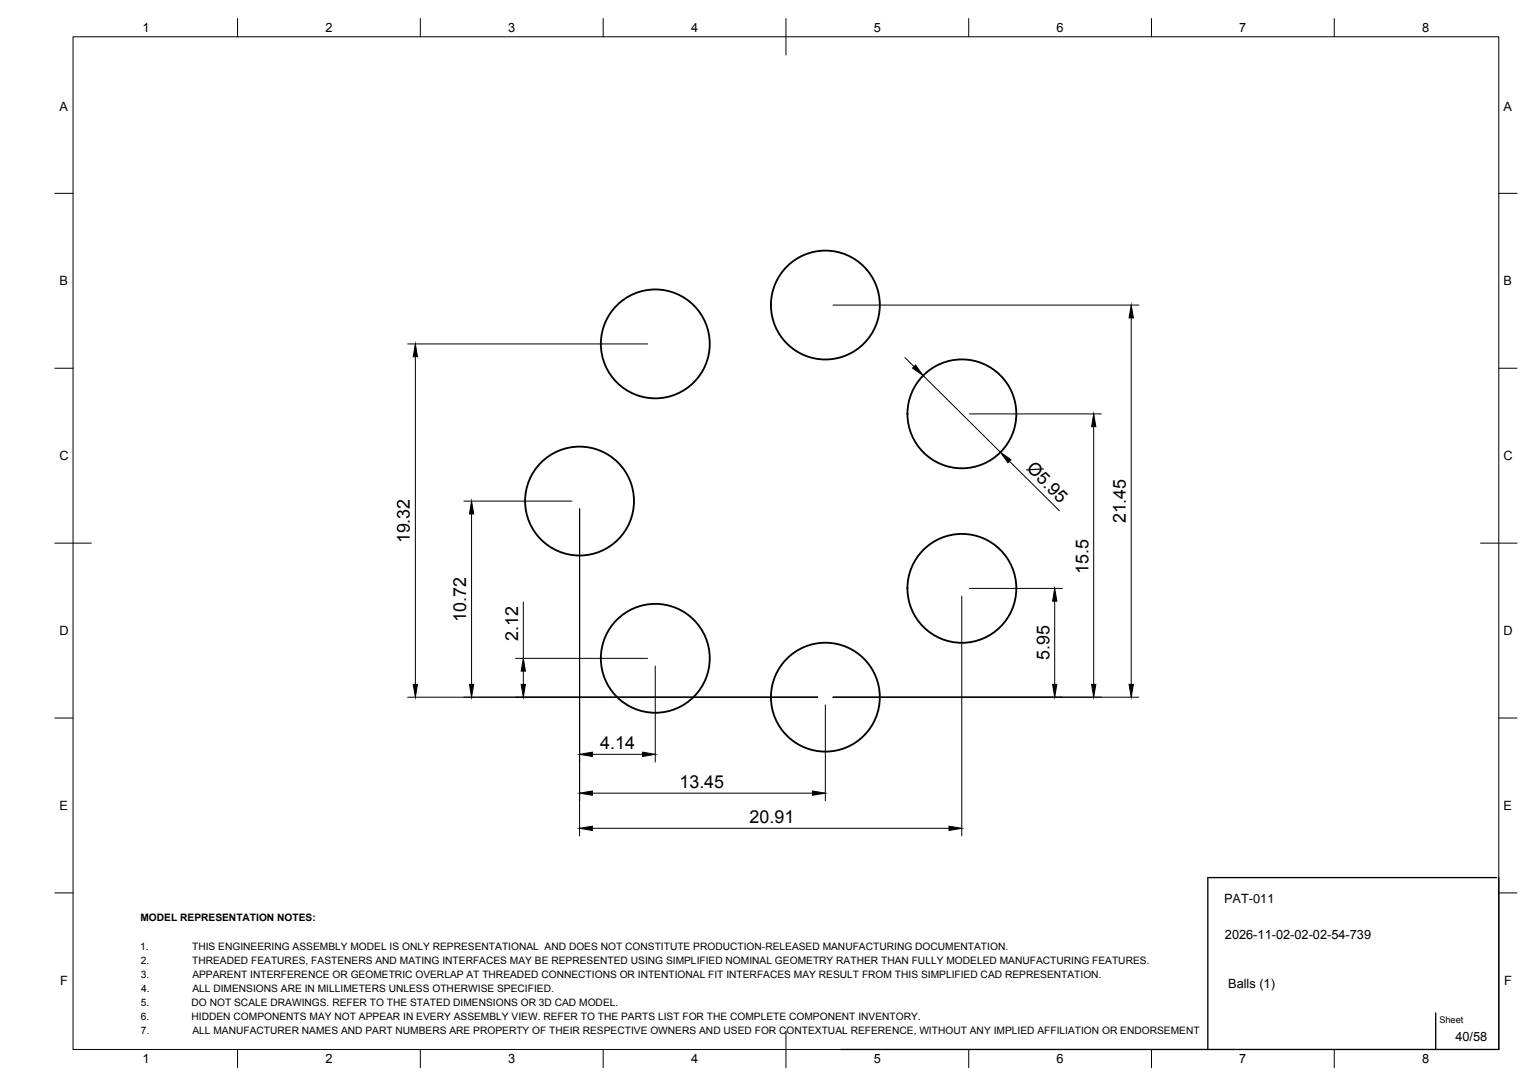
ISO-10303-21;
HEADER;
/* Generated by software containing ST-Developer
 * from STEP Tools, Inc. (www.steptools.com) 
 */

FILE_DESCRIPTION(
/* description */ ('Belt tension measurement rig'),
/* implementation_level */ '2;1');

FILE_NAME(
/* name */ 'Balls (1).step',
/* time_stamp */ '2026-10-28T03:24:44-07:00',
/* author */ (''),
/* organization */ (''),
/* preprocessor_version */ 'ST-DEVELOPER v20.2',
/* originating_system */ 'Autodesk Translation Framework v15.17.0.0',
/* authorisation */ '');

FILE_SCHEMA (('AUTOMOTIVE_DESIGN { 1 0 10303 214 3 1 1 }'));
ENDSEC;

DATA;
#10=MECHANICAL_DESIGN_GEOMETRIC_PRESENTATION_REPRESENTATION('',(#733,#734,#735,#736,#737,#738,#739),#23587);
#453=SPHERICAL_SURFACE('',#13695,0.29765);
#454=SPHERICAL_SURFACE('',#13697,0.29765);
#455=SPHERICAL_SURFACE('',#13699,0.29765);
#456=SPHERICAL_SURFACE('',#13701,0.29765);
#457=SPHERICAL_SURFACE('',#13703,0.29765);
#458=SPHERICAL_SURFACE('',#13705,0.29765);
#459=SPHERICAL_SURFACE('',#13707,0.29765);
#615=SHAPE_REPRESENTATION_RELATIONSHIP('SRR','None',#23864,#670);
#670=ADVANCED_BREP_SHAPE_REPRESENTATION('',(#802,#803,#804,#805,#806,#807,
#808),#23562);
#733=STYLED_ITEM('',(#24211),#802);
#734=STYLED_ITEM('',(#24211),#803);
#735=STYLED_ITEM('',(#24211),#804);
#736=STYLED_ITEM('',(#24211),#805);
#737=STYLED_ITEM('',(#24211),#806);
#738=STYLED_ITEM('',(#24211),#807);
#739=STYLED_ITEM('',(#24211),#808);
#802=MANIFOLD_SOLID_BREP('Body1',#12239);
#803=MANIFOLD_SOLID_BREP('Body2',#12240);
#804=MANIFOLD_SOLID_BREP('Body3',#12241);
#805=MANIFOLD_SOLID_BREP('Body4',#12242);
#806=MANIFOLD_SOLID_BREP('Body5',#12243);
#807=MANIFOLD_SOLID_BREP('Body6',#12244);
#808=MANIFOLD_SOLID_BREP('Body7',#12245);
#1751=FACE_OUTER_BOUND('',#2604,.T.);
#1752=FACE_OUTER_BOUND('',#2605,.T.);
#1753=FACE_OUTER_BOUND('',#2606,.T.);
#1754=FACE_OUTER_BOUND('',#2607,.T.);
#1755=FACE_OUTER_BOUND('',#2608,.T.);
#1756=FACE_OUTER_BOUND('',#2609,.T.);
#1757=FACE_OUTER_BOUND('',#2610,.T.);
#2604=EDGE_LOOP('',(#9726,#9727));
#2605=EDGE_LOOP('',(#9728,#9729));
#2606=EDGE_LOOP('',(#9730,#9731));
#2607=EDGE_LOOP('',(#9732,#9733));
#2608=EDGE_LOOP('',(#9734,#9735));
#2609=EDGE_LOOP('',(#9736,#9737));
#2610=EDGE_LOOP('',(#9738,#9739));
#4842=CIRCLE('',#13696,0.29765);
#4843=CIRCLE('',#13698,0.29765);
#4844=CIRCLE('',#13700,0.29765);
#4845=CIRCLE('',#13702,0.29765);
#4846=CIRCLE('',#13704,0.29765);
#4847=CIRCLE('',#13706,0.29765);
#4848=CIRCLE('',#13708,0.29765);
#5838=VERTEX_POINT('',#20922);
#5839=VERTEX_POINT('',#20923);
#5840=VERTEX_POINT('',#20926);
#5841=VERTEX_POINT('',#20927);
#5842=VERTEX_POINT('',#20930);
#5843=VERTEX_POINT('',#20931);
#5844=VERTEX_POINT('',#20934);
#5845=VERTEX_POINT('',#20935);
#5846=VERTEX_POINT('',#20938);
#5847=VERTEX_POINT('',#20939);
#5848=VERTEX_POINT('',#20942);
#5849=VERTEX_POINT('',#20943);
#5850=VERTEX_POINT('',#20946);
#5851=VERTEX_POINT('',#20947);
#7222=EDGE_CURVE('',#5838,#5839,#4842,.T.);
#7223=EDGE_CURVE('',#5840,#5841,#4843,.T.);
#7224=EDGE_CURVE('',#5842,#5843,#4844,.T.);
#7225=EDGE_CURVE('',#5844,#5845,#4845,.T.);
#7226=EDGE_CURVE('',#5846,#5847,#4846,.T.);
#7227=EDGE_CURVE('',#5848,#5849,#4847,.T.);
#7228=EDGE_CURVE('',#5850,#5851,#4848,.T.);
#9726=ORIENTED_EDGE('',*,*,#7222,.T.);
#9727=ORIENTED_EDGE('',*,*,#7222,.F.);
#9728=ORIENTED_EDGE('',*,*,#7223,.T.);
#9729=ORIENTED_EDGE('',*,*,#7223,.F.);
#9730=ORIENTED_EDGE('',*,*,#7224,.T.);
#9731=ORIENTED_EDGE('',*,*,#7224,.F.);
#9732=ORIENTED_EDGE('',*,*,#7225,.T.);
#9733=ORIENTED_EDGE('',*,*,#7225,.F.);
#9734=ORIENTED_EDGE('',*,*,#7226,.T.);
#9735=ORIENTED_EDGE('',*,*,#7226,.F.);
#9736=ORIENTED_EDGE('',*,*,#7227,.T.);
#9737=ORIENTED_EDGE('',*,*,#7227,.F.);
#9738=ORIENTED_EDGE('',*,*,#7228,.T.);
#9739=ORIENTED_EDGE('',*,*,#7228,.F.);
#11892=ADVANCED_FACE('',(#1751),#453,.T.);
#11893=ADVANCED_FACE('',(#1752),#454,.T.);
#11894=ADVANCED_FACE('',(#1753),#455,.T.);
#11895=ADVANCED_FACE('',(#1754),#456,.T.);
#11896=ADVANCED_FACE('',(#1755),#457,.T.);
#11897=ADVANCED_FACE('',(#1756),#458,.T.);
#11898=ADVANCED_FACE('',(#1757),#459,.T.);
#12239=CLOSED_SHELL('',(#11892));
#12240=CLOSED_SHELL('',(#11893));
#12241=CLOSED_SHELL('',(#11894));
#12242=CLOSED_SHELL('',(#11895));
#12243=CLOSED_SHELL('',(#11896));
#12244=CLOSED_SHELL('',(#11897));
#12245=CLOSED_SHELL('',(#11898));
#13694=AXIS2_PLACEMENT_3D('',#20920,#16649,#16650);
#13695=AXIS2_PLACEMENT_3D('',#20921,#16651,#16652);
#13696=AXIS2_PLACEMENT_3D('',#20924,#16653,#16654);
#13697=AXIS2_PLACEMENT_3D('',#20925,#16655,#16656);
#13698=AXIS2_PLACEMENT_3D('',#20928,#16657,#16658);
#13699=AXIS2_PLACEMENT_3D('',#20929,#16659,#16660);
#13700=AXIS2_PLACEMENT_3D('',#20932,#16661,#16662);
#13701=AXIS2_PLACEMENT_3D('',#20933,#16663,#16664);
#13702=AXIS2_PLACEMENT_3D('',#20936,#16665,#16666);
#13703=AXIS2_PLACEMENT_3D('',#20937,#16667,#16668);
#13704=AXIS2_PLACEMENT_3D('',#20940,#16669,#16670);
#13705=AXIS2_PLACEMENT_3D('',#20941,#16671,#16672);
#13706=AXIS2_PLACEMENT_3D('',#20944,#16673,#16674);
#13707=AXIS2_PLACEMENT_3D('',#20945,#16675,#16676);
#13708=AXIS2_PLACEMENT_3D('',#20948,#16677,#16678);
#16649=DIRECTION('axis',(0.,0.,1.));
#16650=DIRECTION('refdir',(1.,0.,0.));
#16651=DIRECTION('center_axis',(0.,0.,1.));
#16652=DIRECTION('ref_axis',(1.,0.,0.));
#16653=DIRECTION('center_axis',(1.22464679914735E-16,-1.,0.));
#16654=DIRECTION('ref_axis',(-1.,-1.22464679914735E-16,0.));
#16655=DIRECTION('center_axis',(0.78183148246803,0.,0.623489801858733));
#16656=DIRECTION('ref_axis',(0.623489801858734,0.,-0.78183148246803));
#16657=DIRECTION('center_axis',(7.63554790147315E-17,-1.,-9.57467422477103E-17));
#16658=DIRECTION('ref_axis',(-0.623489801858734,-1.22464679914735E-16,0.78183148246803));
#16659=DIRECTION('center_axis',(0.974927912181824,0.,-0.222520933956314));
#16660=DIRECTION('ref_axis',(-0.222520933956314,0.,-0.974927912181824));
#16661=DIRECTION('center_axis',(-2.7250954951288E-17,-1.,-1.19394234705288E-16));
#16662=DIRECTION('ref_axis',(0.222520933956314,-1.22464679914735E-16,0.974927912181824));
#16663=DIRECTION('center_axis',(0.433883739117558,0.,-0.900968867902419));
#16664=DIRECTION('ref_axis',(-0.900968867902419,0.,-0.433883739117558));
#16665=DIRECTION('center_axis',(-1.10336864020811E-16,-1.,-5.31354332312403E-17));
#16666=DIRECTION('ref_axis',(0.900968867902419,-1.22464679914735E-16,0.433883739117558));
#16667=DIRECTION('center_axis',(-0.433883739117558,0.,-0.900968867902419));
#16668=DIRECTION('ref_axis',(-0.900968867902419,0.,0.433883739117558));
#16669=DIRECTION('center_axis',(-1.10336864020811E-16,-1.,5.31354332312403E-17));
#16670=DIRECTION('ref_axis',(0.900968867902419,-1.22464679914735E-16,-0.433883739117558));
#16671=DIRECTION('center_axis',(-0.974927912181824,0.,-0.222520933956314));
#16672=DIRECTION('ref_axis',(-0.222520933956315,0.,0.974927912181824));
#16673=DIRECTION('center_axis',(-2.7250954951288E-17,-1.,1.19394234705288E-16));
#16674=DIRECTION('ref_axis',(0.222520933956315,-1.22464679914735E-16,-0.974927912181824));
#16675=DIRECTION('center_axis',(-0.78183148246803,0.,0.623489801858734));
#16676=DIRECTION('ref_axis',(0.623489801858733,0.,0.78183148246803));
#16677=DIRECTION('center_axis',(7.63554790147315E-17,-1.,9.57467422477103E-17));
#16678=DIRECTION('ref_axis',(-0.623489801858733,-1.22464679914735E-16,-0.78183148246803));
#20920=CARTESIAN_POINT('',(0.,0.,0.));
#20921=CARTESIAN_POINT('Origin',(1.1,0.,0.));
#20922=CARTESIAN_POINT('',(1.1,-2.23201749654651E-33,0.29765));
#20923=CARTESIAN_POINT('',(1.1,-2.23201749654651E-33,-0.29765));
#20924=CARTESIAN_POINT('Origin',(1.1,0.,0.));
#20925=CARTESIAN_POINT('Origin',(0.685838782044607,0.,-0.860014630714833));
#20926=CARTESIAN_POINT('',(0.918550922801216,-5.31350540756609E-33,-0.674432891191581));
#20927=CARTESIAN_POINT('',(0.453126641287998,8.49470414473068E-34,-1.04559637023808));
#20928=CARTESIAN_POINT('Origin',(0.685838782044607,0.,-0.860014630714833));
#20929=CARTESIAN_POINT('Origin',(-0.244773027351946,0.,-1.07242070340001));
#20930=CARTESIAN_POINT('',(0.0454142657089739,-2.23201749654651E-33,-1.1386540593921));
#20931=CARTESIAN_POINT('',(-0.534960320412865,-2.23201749654651E-33,-1.00618734740791));
#20932=CARTESIAN_POINT('Origin',(-0.244773027351946,0.,-1.07242070340001));
#20933=CARTESIAN_POINT('Origin',(-0.991065754692661,0.,-0.477272113029314));
#20934=CARTESIAN_POINT('',(-0.86192025974432,8.49470414473067E-34,-0.745445496560469));
#20935=CARTESIAN_POINT('',(-1.120211249641,-5.31350540756609E-33,-0.209098729498159));
#20936=CARTESIAN_POINT('Origin',(-0.991065754692661,0.,-0.477272113029314));
#20937=CARTESIAN_POINT('Origin',(-0.991065754692661,0.,0.477272113029314));
#20938=CARTESIAN_POINT('',(-1.120211249641,-2.23201749654651E-33,0.209098729498159));
#20939=CARTESIAN_POINT('',(-0.86192025974432,-2.23201749654651E-33,0.745445496560469));
#20940=CARTESIAN_POINT('Origin',(-0.991065754692661,0.,0.477272113029314));
#20941=CARTESIAN_POINT('Origin',(-0.244773027351946,0.,1.07242070340001));
#20942=CARTESIAN_POINT('',(-0.534960320412866,-2.23201749654651E-33,1.00618734740791));
#20943=CARTESIAN_POINT('',(0.0454142657089737,-2.23201749654651E-33,1.1386540593921));
#20944=CARTESIAN_POINT('Origin',(-0.244773027351946,0.,1.07242070340001));
#20945=CARTESIAN_POINT('Origin',(0.685838782044607,0.,0.860014630714833));
#20946=CARTESIAN_POINT('',(0.453126641287998,-2.23201749654651E-33,1.04559637023808));
#20947=CARTESIAN_POINT('',(0.918550922801216,-2.23201749654651E-33,0.674432891191581));
#20948=CARTESIAN_POINT('Origin',(0.685838782044607,0.,0.860014630714833));
#23497=UNCERTAINTY_MEASURE_WITH_UNIT(LENGTH_MEASURE(0.001),#23588,
'DISTANCE_ACCURACY_VALUE',
'Maximum model space distance between geometric entities at asserted c
onnectivities');
#23522=UNCERTAINTY_MEASURE_WITH_UNIT(LENGTH_MEASURE(0.001),#23588,
'DISTANCE_ACCURACY_VALUE',
'Maximum model space distance between geometric entities at asserted c
onnectivities');
#23562=(
GEOMETRIC_REPRESENTATION_CONTEXT(3)
GLOBAL_UNCERTAINTY_ASSIGNED_CONTEXT((#23497))
GLOBAL_UNIT_ASSIGNED_CONTEXT((#23588,#23590,#23591))
REPRESENTATION_CONTEXT('','3D')
);
#23587=(
GEOMETRIC_REPRESENTATION_CONTEXT(3)
GLOBAL_UNCERTAINTY_ASSIGNED_CONTEXT((#23522))
GLOBAL_UNIT_ASSIGNED_CONTEXT((#23588,#23590,#23591))
REPRESENTATION_CONTEXT('','3D')
);
#23588=(
LENGTH_UNIT()
NAMED_UNIT(*)
SI_UNIT(.CENTI.,.METRE.)
);
#23590=(
NAMED_UNIT(*)
PLANE_ANGLE_UNIT()
SI_UNIT($,.RADIAN.)
);
#23591=(
NAMED_UNIT(*)
SI_UNIT($,.STERADIAN.)
SOLID_ANGLE_UNIT()
);
#23631=SHAPE_DEFINITION_REPRESENTATION(#23703,#23864);
#23703=PRODUCT_DEFINITION_SHAPE('',$,#23929);
#23864=SHAPE_REPRESENTATION('',(#13694),#23562);
#23889=PRODUCT_DEFINITION_CONTEXT('part definition',#24083,'design');
#23929=PRODUCT_DEFINITION('Balls (1)','Balls (1)',#23993,#23889);
#23993=PRODUCT_DEFINITION_FORMATION('',$,#24124);
#24083=APPLICATION_CONTEXT(
'Core Data for Automotive Mechanical Design Process');
#24084=PRODUCT_CONTEXT('part definition',#24083,'mechanical');
#24124=PRODUCT('Balls (1)','Balls (1)','Balls (1)',(#24084));
#24205=COLOUR_RGB('Grey',0.48,0.52,0.57);
#24206=FILL_AREA_STYLE_COLOUR('',#24205);
#24207=FILL_AREA_STYLE('',(#24206));
#24208=SURFACE_STYLE_FILL_AREA(#24207);
#24209=SURFACE_SIDE_STYLE('',(#24208));
#24210=SURFACE_STYLE_USAGE(.BOTH.,#24209);
#24211=PRESENTATION_STYLE_ASSIGNMENT((#24210));
ENDSEC;
END-ISO-10303-21;
